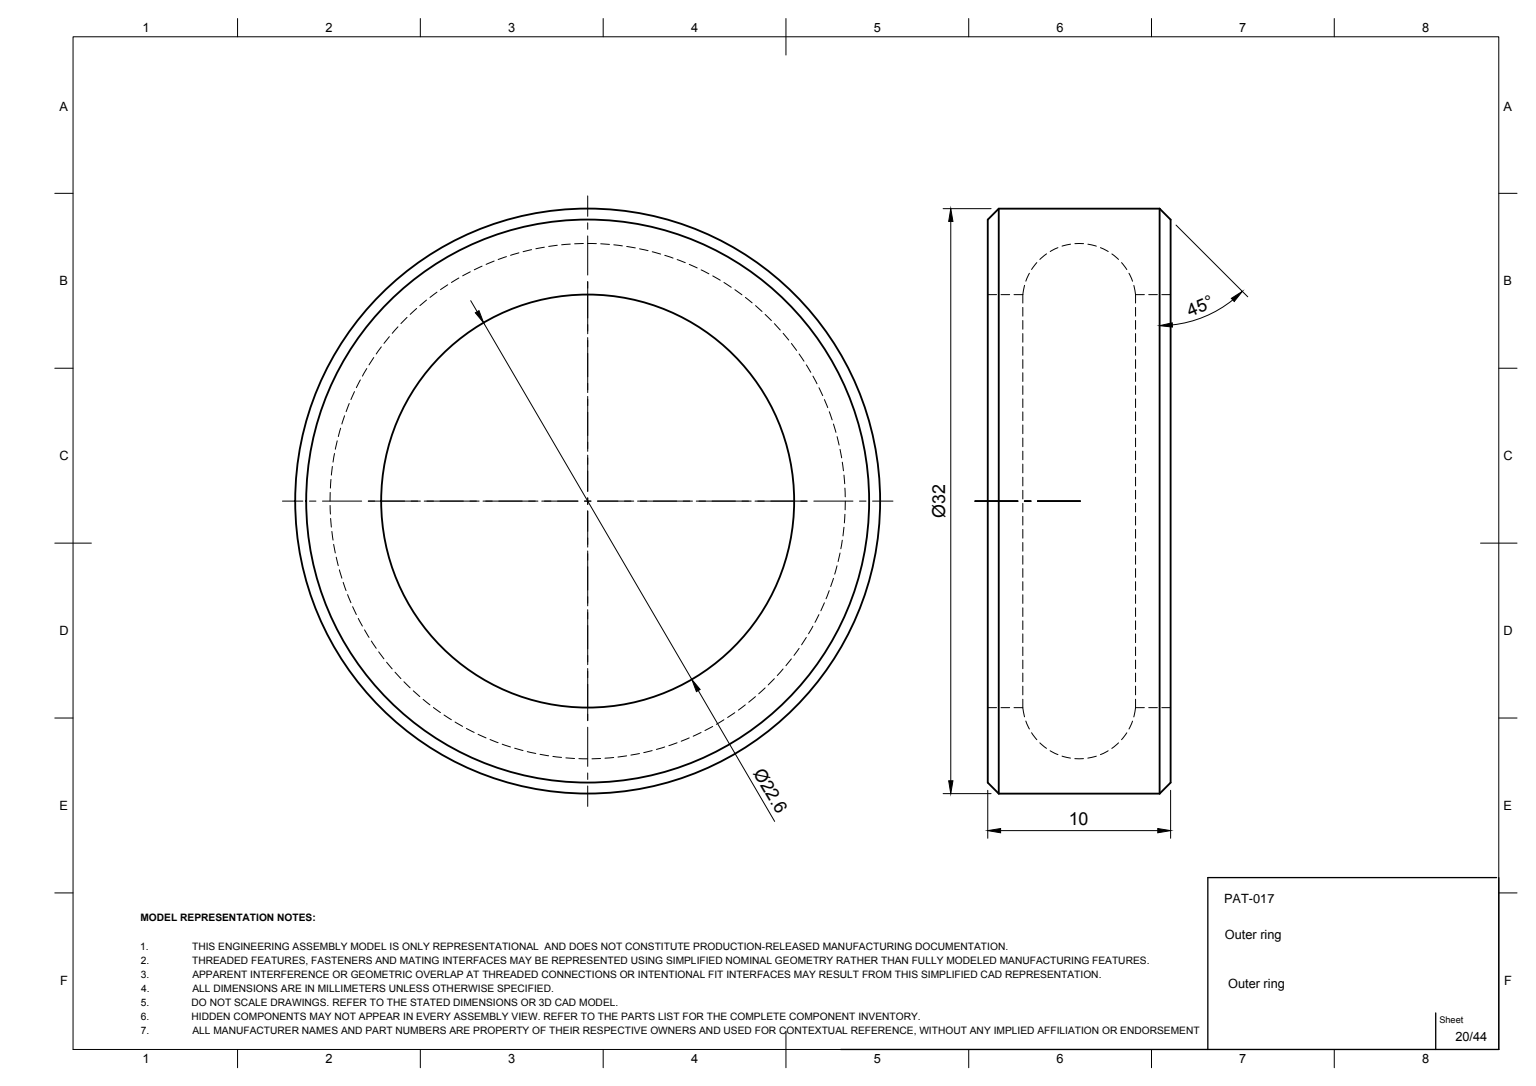
ISO-10303-21;
HEADER;
/* Generated by software containing ST-Developer
 * from STEP Tools, Inc. (www.steptools.com) 
 */

FILE_DESCRIPTION(
/* description */ ('Cam-and-follower valve demonstrator'),
/* implementation_level */ '2;1');

FILE_NAME(
/* name */ 'Outer ring.step',
/* time_stamp */ '2026-10-28T03:25:17-07:00',
/* author */ (''),
/* organization */ (''),
/* preprocessor_version */ 'ST-DEVELOPER v20.2',
/* originating_system */ 'Autodesk Translation Framework v15.17.0.0',
/* authorisation */ '');

FILE_SCHEMA (('AUTOMOTIVE_DESIGN { 1 0 10303 214 3 1 1 }'));
ENDSEC;

DATA;
#10=MECHANICAL_DESIGN_GEOMETRIC_PRESENTATION_REPRESENTATION('',(#425),#12896);
#309=CONICAL_SURFACE('',#6947,1.57,0.785398163397449);
#310=CONICAL_SURFACE('',#6951,1.57,0.785398163397449);
#323=TOROIDAL_SURFACE('',#6936,1.1,0.309556);
#353=SHAPE_REPRESENTATION_RELATIONSHIP('SRR','None',#13070,#389);
#389=ADVANCED_BREP_SHAPE_REPRESENTATION('',(#468),#12870);
#425=STYLED_ITEM('',(#13330),#468);
#468=MANIFOLD_SOLID_BREP('Body1',#6192);
#606=FACE_BOUND('',#1732,.T.);
#607=FACE_BOUND('',#1737,.T.);
#802=CIRCLE('',#6937,1.129765);
#803=CIRCLE('',#6938,1.129765);
#804=CIRCLE('',#6939,0.309556);
#805=CIRCLE('',#6940,1.129765);
#806=CIRCLE('',#6941,1.129765);
#807=CIRCLE('',#6943,1.129765);
#808=CIRCLE('',#6945,1.54);
#809=CIRCLE('',#6946,1.129765);
#810=CIRCLE('',#6948,1.6);
#811=CIRCLE('',#6950,1.6);
#812=CIRCLE('',#6952,1.54);
#1041=CYLINDRICAL_SURFACE('',#6942,1.129765);
#1042=CYLINDRICAL_SURFACE('',#6949,1.6);
#1043=CYLINDRICAL_SURFACE('',#6954,1.129765);
#1250=FACE_OUTER_BOUND('',#1729,.T.);
#1251=FACE_OUTER_BOUND('',#1730,.T.);
#1252=FACE_OUTER_BOUND('',#1731,.T.);
#1253=FACE_OUTER_BOUND('',#1733,.T.);
#1254=FACE_OUTER_BOUND('',#1734,.T.);
#1255=FACE_OUTER_BOUND('',#1735,.T.);
#1256=FACE_OUTER_BOUND('',#1736,.T.);
#1257=FACE_OUTER_BOUND('',#1738,.T.);
#1729=EDGE_LOOP('',(#4787,#4788,#4789,#4790,#4791,#4792));
#1730=EDGE_LOOP('',(#4793,#4794,#4795,#4796,#4797));
#1731=EDGE_LOOP('',(#4798));
#1732=EDGE_LOOP('',(#4799));
#1733=EDGE_LOOP('',(#4800,#4801,#4802,#4803));
#1734=EDGE_LOOP('',(#4804,#4805,#4806,#4807));
#1735=EDGE_LOOP('',(#4808,#4809,#4810,#4811));
#1736=EDGE_LOOP('',(#4812));
#1737=EDGE_LOOP('',(#4813));
#1738=EDGE_LOOP('',(#4814,#4815,#4816,#4817,#4818));
#2197=LINE('',#11543,#2619);
#2198=LINE('',#11552,#2620);
#2199=LINE('',#11556,#2621);
#2200=LINE('',#11560,#2622);
#2201=LINE('',#11563,#2623);
#2619=VECTOR('',#8260,1.129765);
#2620=VECTOR('',#8271,1.57);
#2621=VECTOR('',#8276,1.6);
#2622=VECTOR('',#8281,1.57);
#2623=VECTOR('',#8286,1.129765);
#3069=VERTEX_POINT('',#11531);
#3070=VERTEX_POINT('',#11532);
#3071=VERTEX_POINT('',#11535);
#3072=VERTEX_POINT('',#11537);
#3073=VERTEX_POINT('',#11541);
#3074=VERTEX_POINT('',#11545);
#3075=VERTEX_POINT('',#11547);
#3076=VERTEX_POINT('',#11550);
#3077=VERTEX_POINT('',#11554);
#3078=VERTEX_POINT('',#11558);
#3690=EDGE_CURVE('',#3069,#3070,#802,.T.);
#3691=EDGE_CURVE('',#3070,#3069,#803,.T.);
#3692=EDGE_CURVE('',#3070,#3071,#804,.T.);
#3693=EDGE_CURVE('',#3072,#3071,#805,.T.);
#3694=EDGE_CURVE('',#3071,#3072,#806,.T.);
#3695=EDGE_CURVE('',#3073,#3073,#807,.T.);
#3696=EDGE_CURVE('',#3073,#3072,#2197,.T.);
#3697=EDGE_CURVE('',#3074,#3074,#808,.T.);
#3698=EDGE_CURVE('',#3075,#3075,#809,.T.);
#3699=EDGE_CURVE('',#3076,#3076,#810,.T.);
#3700=EDGE_CURVE('',#3076,#3074,#2198,.T.);
#3701=EDGE_CURVE('',#3077,#3077,#811,.T.);
#3702=EDGE_CURVE('',#3077,#3076,#2199,.T.);
#3703=EDGE_CURVE('',#3078,#3078,#812,.T.);
#3704=EDGE_CURVE('',#3078,#3077,#2200,.T.);
#3705=EDGE_CURVE('',#3069,#3075,#2201,.T.);
#4787=ORIENTED_EDGE('',*,*,#3690,.F.);
#4788=ORIENTED_EDGE('',*,*,#3691,.F.);
#4789=ORIENTED_EDGE('',*,*,#3692,.T.);
#4790=ORIENTED_EDGE('',*,*,#3693,.F.);
#4791=ORIENTED_EDGE('',*,*,#3694,.F.);
#4792=ORIENTED_EDGE('',*,*,#3692,.F.);
#4793=ORIENTED_EDGE('',*,*,#3695,.T.);
#4794=ORIENTED_EDGE('',*,*,#3696,.T.);
#4795=ORIENTED_EDGE('',*,*,#3693,.T.);
#4796=ORIENTED_EDGE('',*,*,#3694,.T.);
#4797=ORIENTED_EDGE('',*,*,#3696,.F.);
#4798=ORIENTED_EDGE('',*,*,#3697,.F.);
#4799=ORIENTED_EDGE('',*,*,#3698,.T.);
#4800=ORIENTED_EDGE('',*,*,#3699,.F.);
#4801=ORIENTED_EDGE('',*,*,#3700,.T.);
#4802=ORIENTED_EDGE('',*,*,#3697,.T.);
#4803=ORIENTED_EDGE('',*,*,#3700,.F.);
#4804=ORIENTED_EDGE('',*,*,#3701,.F.);
#4805=ORIENTED_EDGE('',*,*,#3702,.T.);
#4806=ORIENTED_EDGE('',*,*,#3699,.T.);
#4807=ORIENTED_EDGE('',*,*,#3702,.F.);
#4808=ORIENTED_EDGE('',*,*,#3703,.F.);
#4809=ORIENTED_EDGE('',*,*,#3704,.T.);
#4810=ORIENTED_EDGE('',*,*,#3701,.T.);
#4811=ORIENTED_EDGE('',*,*,#3704,.F.);
#4812=ORIENTED_EDGE('',*,*,#3703,.T.);
#4813=ORIENTED_EDGE('',*,*,#3695,.F.);
#4814=ORIENTED_EDGE('',*,*,#3690,.T.);
#4815=ORIENTED_EDGE('',*,*,#3691,.T.);
#4816=ORIENTED_EDGE('',*,*,#3705,.T.);
#4817=ORIENTED_EDGE('',*,*,#3698,.F.);
#4818=ORIENTED_EDGE('',*,*,#3705,.F.);
#5680=PLANE('',#6944);
#5681=PLANE('',#6953);
#5966=ADVANCED_FACE('',(#1250),#323,.F.);
#5967=ADVANCED_FACE('',(#1251),#1041,.F.);
#5968=ADVANCED_FACE('',(#1252,#606),#5680,.T.);
#5969=ADVANCED_FACE('',(#1253),#309,.T.);
#5970=ADVANCED_FACE('',(#1254),#1042,.T.);
#5971=ADVANCED_FACE('',(#1255),#310,.T.);
#5972=ADVANCED_FACE('',(#1256,#607),#5681,.T.);
#5973=ADVANCED_FACE('',(#1257),#1043,.F.);
#6192=CLOSED_SHELL('',(#5966,#5967,#5968,#5969,#5970,#5971,#5972,#5973));
#6935=AXIS2_PLACEMENT_3D('',#11529,#8242,#8243);
#6936=AXIS2_PLACEMENT_3D('',#11530,#8244,#8245);
#6937=AXIS2_PLACEMENT_3D('',#11533,#8246,#8247);
#6938=AXIS2_PLACEMENT_3D('',#11534,#8248,#8249);
#6939=AXIS2_PLACEMENT_3D('',#11536,#8250,#8251);
#6940=AXIS2_PLACEMENT_3D('',#11538,#8252,#8253);
#6941=AXIS2_PLACEMENT_3D('',#11539,#8254,#8255);
#6942=AXIS2_PLACEMENT_3D('',#11540,#8256,#8257);
#6943=AXIS2_PLACEMENT_3D('',#11542,#8258,#8259);
#6944=AXIS2_PLACEMENT_3D('',#11544,#8261,#8262);
#6945=AXIS2_PLACEMENT_3D('',#11546,#8263,#8264);
#6946=AXIS2_PLACEMENT_3D('',#11548,#8265,#8266);
#6947=AXIS2_PLACEMENT_3D('',#11549,#8267,#8268);
#6948=AXIS2_PLACEMENT_3D('',#11551,#8269,#8270);
#6949=AXIS2_PLACEMENT_3D('',#11553,#8272,#8273);
#6950=AXIS2_PLACEMENT_3D('',#11555,#8274,#8275);
#6951=AXIS2_PLACEMENT_3D('',#11557,#8277,#8278);
#6952=AXIS2_PLACEMENT_3D('',#11559,#8279,#8280);
#6953=AXIS2_PLACEMENT_3D('',#11561,#8282,#8283);
#6954=AXIS2_PLACEMENT_3D('',#11562,#8284,#8285);
#8242=DIRECTION('axis',(0.,0.,1.));
#8243=DIRECTION('refdir',(1.,0.,0.));
#8244=DIRECTION('center_axis',(0.,-1.,0.));
#8245=DIRECTION('ref_axis',(0.,0.,-1.));
#8246=DIRECTION('center_axis',(0.,-1.,0.));
#8247=DIRECTION('ref_axis',(1.,0.,0.));
#8248=DIRECTION('center_axis',(0.,-1.,0.));
#8249=DIRECTION('ref_axis',(1.,0.,0.));
#8250=DIRECTION('center_axis',(1.,0.,1.22464679914735E-16));
#8251=DIRECTION('ref_axis',(-1.22464679914735E-16,0.,1.));
#8252=DIRECTION('center_axis',(0.,1.,0.));
#8253=DIRECTION('ref_axis',(1.,0.,0.));
#8254=DIRECTION('center_axis',(0.,1.,0.));
#8255=DIRECTION('ref_axis',(1.,0.,0.));
#8256=DIRECTION('center_axis',(0.,-1.,0.));
#8257=DIRECTION('ref_axis',(1.,0.,0.));
#8258=DIRECTION('center_axis',(0.,-1.,0.));
#8259=DIRECTION('ref_axis',(1.,0.,0.));
#8260=DIRECTION('',(0.,1.,0.));
#8261=DIRECTION('center_axis',(0.,1.,0.));
#8262=DIRECTION('ref_axis',(0.,0.,1.));
#8263=DIRECTION('center_axis',(0.,-1.,0.));
#8264=DIRECTION('ref_axis',(1.,0.,0.));
#8265=DIRECTION('center_axis',(0.,-1.,0.));
#8266=DIRECTION('ref_axis',(1.,0.,0.));
#8267=DIRECTION('center_axis',(0.,-1.,0.));
#8268=DIRECTION('ref_axis',(1.,0.,0.));
#8269=DIRECTION('center_axis',(0.,-1.,0.));
#8270=DIRECTION('ref_axis',(1.,0.,0.));
#8271=DIRECTION('',(0.707106781186548,0.707106781186547,8.65956056235494E-17));
#8272=DIRECTION('center_axis',(0.,-1.,0.));
#8273=DIRECTION('ref_axis',(1.,0.,0.));
#8274=DIRECTION('center_axis',(0.,-1.,0.));
#8275=DIRECTION('ref_axis',(1.,0.,0.));
#8276=DIRECTION('',(0.,1.,0.));
#8277=DIRECTION('center_axis',(0.,1.,0.));
#8278=DIRECTION('ref_axis',(1.,0.,0.));
#8279=DIRECTION('center_axis',(0.,-1.,0.));
#8280=DIRECTION('ref_axis',(1.,0.,0.));
#8281=DIRECTION('',(-0.707106781186548,0.707106781186547,-8.65956056235494E-17));
#8282=DIRECTION('center_axis',(0.,-1.,0.));
#8283=DIRECTION('ref_axis',(0.,0.,-1.));
#8284=DIRECTION('center_axis',(0.,-1.,0.));
#8285=DIRECTION('ref_axis',(1.,0.,0.));
#8286=DIRECTION('',(0.,1.,0.));
#11529=CARTESIAN_POINT('',(0.,0.,0.));
#11530=CARTESIAN_POINT('Origin',(0.,0.,0.));
#11531=CARTESIAN_POINT('',(-1.129765,0.308121667383195,-1.38356309103871E-16));
#11532=CARTESIAN_POINT('',(-1.38356309103871E-16,0.308121667383195,1.129765));
#11533=CARTESIAN_POINT('Origin',(0.,0.308121667383195,0.));
#11534=CARTESIAN_POINT('Origin',(0.,0.308121667383195,0.));
#11535=CARTESIAN_POINT('',(-1.38356309103871E-16,-0.308121667383195,1.129765));
#11536=CARTESIAN_POINT('Origin',(-1.34711147906209E-16,0.,1.1));
#11537=CARTESIAN_POINT('',(-1.129765,-0.308121667383195,1.38356309103871E-16));
#11538=CARTESIAN_POINT('Origin',(0.,-0.308121667383195,0.));
#11539=CARTESIAN_POINT('Origin',(0.,-0.308121667383195,0.));
#11540=CARTESIAN_POINT('Origin',(0.,0.,0.));
#11541=CARTESIAN_POINT('',(-1.129765,-0.5,-1.38356309103871E-16));
#11542=CARTESIAN_POINT('Origin',(0.,-0.5,0.));
#11543=CARTESIAN_POINT('',(-1.129765,0.,-1.38356309103871E-16));
#11544=CARTESIAN_POINT('Origin',(1.54,0.5,0.));
#11545=CARTESIAN_POINT('',(-1.54,0.5,-1.88595607068692E-16));
#11546=CARTESIAN_POINT('Origin',(0.,0.5,0.));
#11547=CARTESIAN_POINT('',(-1.129765,0.5,-1.38356309103871E-16));
#11548=CARTESIAN_POINT('Origin',(0.,0.5,0.));
#11549=CARTESIAN_POINT('Origin',(0.,0.47,0.));
#11550=CARTESIAN_POINT('',(-1.6,0.44,-1.95943487863577E-16));
#11551=CARTESIAN_POINT('Origin',(0.,0.44,0.));
#11552=CARTESIAN_POINT('',(-1.57,0.47,-1.92269547466134E-16));
#11553=CARTESIAN_POINT('Origin',(0.,0.,0.));
#11554=CARTESIAN_POINT('',(-1.6,-0.44,-1.95943487863577E-16));
#11555=CARTESIAN_POINT('Origin',(0.,-0.44,0.));
#11556=CARTESIAN_POINT('',(-1.6,0.,-1.95943487863577E-16));
#11557=CARTESIAN_POINT('Origin',(0.,-0.47,0.));
#11558=CARTESIAN_POINT('',(-1.54,-0.5,-1.88595607068692E-16));
#11559=CARTESIAN_POINT('Origin',(0.,-0.5,0.));
#11560=CARTESIAN_POINT('',(-1.57,-0.47,-1.92269547466134E-16));
#11561=CARTESIAN_POINT('Origin',(1.129765,-0.5,0.));
#11562=CARTESIAN_POINT('Origin',(0.,0.,0.));
#11563=CARTESIAN_POINT('',(-1.129765,0.,-1.38356309103871E-16));
#12827=UNCERTAINTY_MEASURE_WITH_UNIT(LENGTH_MEASURE(0.001),#12897,
'DISTANCE_ACCURACY_VALUE',
'Maximum model space distance between geometric entities at asserted c
onnectivities');
#12853=UNCERTAINTY_MEASURE_WITH_UNIT(LENGTH_MEASURE(0.001),#12897,
'DISTANCE_ACCURACY_VALUE',
'Maximum model space distance between geometric entities at asserted c
onnectivities');
#12870=(
GEOMETRIC_REPRESENTATION_CONTEXT(3)
GLOBAL_UNCERTAINTY_ASSIGNED_CONTEXT((#12827))
GLOBAL_UNIT_ASSIGNED_CONTEXT((#12897,#12899,#12900))
REPRESENTATION_CONTEXT('','3D')
);
#12896=(
GEOMETRIC_REPRESENTATION_CONTEXT(3)
GLOBAL_UNCERTAINTY_ASSIGNED_CONTEXT((#12853))
GLOBAL_UNIT_ASSIGNED_CONTEXT((#12897,#12899,#12900))
REPRESENTATION_CONTEXT('','3D')
);
#12897=(
LENGTH_UNIT()
NAMED_UNIT(*)
SI_UNIT(.CENTI.,.METRE.)
);
#12899=(
NAMED_UNIT(*)
PLANE_ANGLE_UNIT()
SI_UNIT($,.RADIAN.)
);
#12900=(
NAMED_UNIT(*)
SI_UNIT($,.STERADIAN.)
SOLID_ANGLE_UNIT()
);
#12917=SHAPE_DEFINITION_REPRESENTATION(#12959,#13070);
#12959=PRODUCT_DEFINITION_SHAPE('',$,#13113);
#13070=SHAPE_REPRESENTATION('',(#6935),#12870);
#13096=PRODUCT_DEFINITION_CONTEXT('part definition',#13224,'design');
#13113=PRODUCT_DEFINITION('Outer ring','Outer ring',#13155,#13096);
#13155=PRODUCT_DEFINITION_FORMATION('',$,#13242);
#13224=APPLICATION_CONTEXT(
'Core Data for Automotive Mechanical Design Process');
#13225=PRODUCT_CONTEXT('part definition',#13224,'mechanical');
#13242=PRODUCT('Outer ring','Outer ring','Outer ring',(#13225));
#13324=COLOUR_RGB('Grey',0.48,0.52,0.57);
#13325=FILL_AREA_STYLE_COLOUR('',#13324);
#13326=FILL_AREA_STYLE('',(#13325));
#13327=SURFACE_STYLE_FILL_AREA(#13326);
#13328=SURFACE_SIDE_STYLE('',(#13327));
#13329=SURFACE_STYLE_USAGE(.BOTH.,#13328);
#13330=PRESENTATION_STYLE_ASSIGNMENT((#13329));
ENDSEC;
END-ISO-10303-21;
